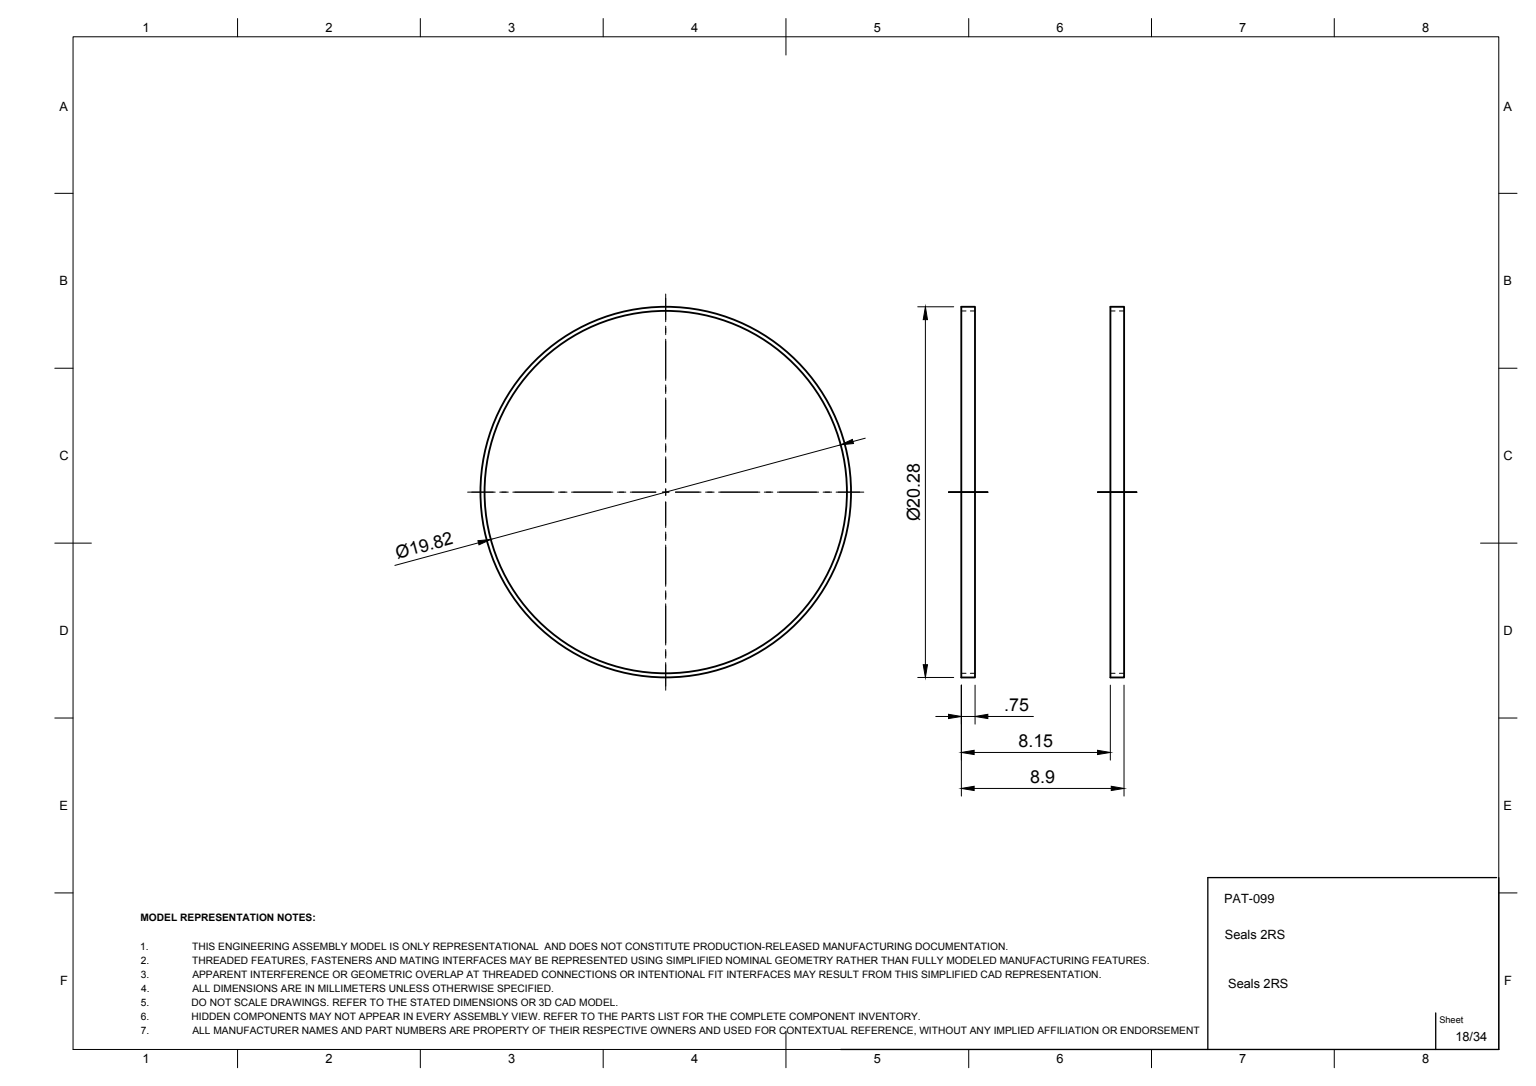
ISO-10303-21;
HEADER;
/* Generated by software containing ST-Developer
 * from STEP Tools, Inc. (www.steptools.com) 
 */

FILE_DESCRIPTION(
/* description */ ('PAT-099'),
/* implementation_level */ '2;1');

FILE_NAME(
/* name */ 'Seals 2RS.step',
/* time_stamp */ '2026-10-29T17:25:42-07:00',
/* author */ (''),
/* organization */ (''),
/* preprocessor_version */ 'ST-DEVELOPER v20.2',
/* originating_system */ 'Autodesk Translation Framework v15.17.0.0',
/* authorisation */ '');

FILE_SCHEMA (('AUTOMOTIVE_DESIGN { 1 0 10303 214 3 1 1 }'));
ENDSEC;

DATA;
#10=MECHANICAL_DESIGN_GEOMETRIC_PRESENTATION_REPRESENTATION('',(#368,#369),#11035);
#311=SHAPE_REPRESENTATION_RELATIONSHIP('SRR','None',#11184,#336);
#336=ADVANCED_BREP_SHAPE_REPRESENTATION('',(#399,#400),#11034);
#368=STYLED_ITEM('',(#11386),#399);
#369=STYLED_ITEM('',(#11386),#400);
#399=MANIFOLD_SOLID_BREP('Body1',#4738);
#400=MANIFOLD_SOLID_BREP('Body2',#4739);
#519=FACE_BOUND('',#1332,.T.);
#520=FACE_BOUND('',#1335,.T.);
#521=FACE_BOUND('',#1338,.T.);
#522=FACE_BOUND('',#1341,.T.);
#655=PLANE('',#5615);
#656=PLANE('',#5620);
#657=PLANE('',#5623);
#658=PLANE('',#5628);
#932=FACE_OUTER_BOUND('',#1331,.T.);
#933=FACE_OUTER_BOUND('',#1333,.T.);
#934=FACE_OUTER_BOUND('',#1334,.T.);
#935=FACE_OUTER_BOUND('',#1336,.T.);
#936=FACE_OUTER_BOUND('',#1337,.T.);
#937=FACE_OUTER_BOUND('',#1339,.T.);
#938=FACE_OUTER_BOUND('',#1340,.T.);
#939=FACE_OUTER_BOUND('',#1342,.T.);
#1331=EDGE_LOOP('',(#4285));
#1332=EDGE_LOOP('',(#4286));
#1333=EDGE_LOOP('',(#4287,#4288,#4289,#4290));
#1334=EDGE_LOOP('',(#4291));
#1335=EDGE_LOOP('',(#4292));
#1336=EDGE_LOOP('',(#4293,#4294,#4295,#4296));
#1337=EDGE_LOOP('',(#4297));
#1338=EDGE_LOOP('',(#4298));
#1339=EDGE_LOOP('',(#4299,#4300,#4301,#4302));
#1340=EDGE_LOOP('',(#4303));
#1341=EDGE_LOOP('',(#4304));
#1342=EDGE_LOOP('',(#4305,#4306,#4307,#4308));
#1591=LINE('',#10913,#1843);
#1592=LINE('',#10918,#1844);
#1593=LINE('',#10927,#1845);
#1594=LINE('',#10932,#1846);
#1843=VECTOR('',#7124,1.013815);
#1844=VECTOR('',#7131,0.991185);
#1845=VECTOR('',#7142,1.013815);
#1846=VECTOR('',#7149,0.991185);
#2130=CIRCLE('',#5616,1.013815);
#2131=CIRCLE('',#5617,0.991185);
#2132=CIRCLE('',#5619,1.013815);
#2133=CIRCLE('',#5621,0.991185);
#2134=CIRCLE('',#5624,1.013815);
#2135=CIRCLE('',#5625,0.991185);
#2136=CIRCLE('',#5627,1.013815);
#2137=CIRCLE('',#5629,0.991185);
#2534=VERTEX_POINT('',#10906);
#2535=VERTEX_POINT('',#10908);
#2536=VERTEX_POINT('',#10911);
#2537=VERTEX_POINT('',#10915);
#2538=VERTEX_POINT('',#10920);
#2539=VERTEX_POINT('',#10922);
#2540=VERTEX_POINT('',#10925);
#2541=VERTEX_POINT('',#10929);
#3119=EDGE_CURVE('',#2534,#2534,#2130,.T.);
#3120=EDGE_CURVE('',#2535,#2535,#2131,.T.);
#3121=EDGE_CURVE('',#2536,#2536,#2132,.T.);
#3122=EDGE_CURVE('',#2536,#2534,#1591,.T.);
#3123=EDGE_CURVE('',#2537,#2537,#2133,.T.);
#3124=EDGE_CURVE('',#2537,#2535,#1592,.T.);
#3125=EDGE_CURVE('',#2538,#2538,#2134,.T.);
#3126=EDGE_CURVE('',#2539,#2539,#2135,.T.);
#3127=EDGE_CURVE('',#2540,#2540,#2136,.T.);
#3128=EDGE_CURVE('',#2540,#2538,#1593,.T.);
#3129=EDGE_CURVE('',#2541,#2541,#2137,.T.);
#3130=EDGE_CURVE('',#2541,#2539,#1594,.T.);
#4285=ORIENTED_EDGE('',*,*,#3119,.F.);
#4286=ORIENTED_EDGE('',*,*,#3120,.T.);
#4287=ORIENTED_EDGE('',*,*,#3121,.F.);
#4288=ORIENTED_EDGE('',*,*,#3122,.T.);
#4289=ORIENTED_EDGE('',*,*,#3119,.T.);
#4290=ORIENTED_EDGE('',*,*,#3122,.F.);
#4291=ORIENTED_EDGE('',*,*,#3121,.T.);
#4292=ORIENTED_EDGE('',*,*,#3123,.F.);
#4293=ORIENTED_EDGE('',*,*,#3123,.T.);
#4294=ORIENTED_EDGE('',*,*,#3124,.T.);
#4295=ORIENTED_EDGE('',*,*,#3120,.F.);
#4296=ORIENTED_EDGE('',*,*,#3124,.F.);
#4297=ORIENTED_EDGE('',*,*,#3125,.F.);
#4298=ORIENTED_EDGE('',*,*,#3126,.T.);
#4299=ORIENTED_EDGE('',*,*,#3127,.F.);
#4300=ORIENTED_EDGE('',*,*,#3128,.T.);
#4301=ORIENTED_EDGE('',*,*,#3125,.T.);
#4302=ORIENTED_EDGE('',*,*,#3128,.F.);
#4303=ORIENTED_EDGE('',*,*,#3127,.T.);
#4304=ORIENTED_EDGE('',*,*,#3129,.F.);
#4305=ORIENTED_EDGE('',*,*,#3129,.T.);
#4306=ORIENTED_EDGE('',*,*,#3130,.T.);
#4307=ORIENTED_EDGE('',*,*,#3126,.F.);
#4308=ORIENTED_EDGE('',*,*,#3130,.F.);
#4420=CYLINDRICAL_SURFACE('',#5618,1.013815);
#4421=CYLINDRICAL_SURFACE('',#5622,0.991185);
#4422=CYLINDRICAL_SURFACE('',#5626,1.013815);
#4423=CYLINDRICAL_SURFACE('',#5630,0.991185);
#4697=ADVANCED_FACE('',(#932,#519),#655,.T.);
#4698=ADVANCED_FACE('',(#933),#4420,.T.);
#4699=ADVANCED_FACE('',(#934,#520),#656,.T.);
#4700=ADVANCED_FACE('',(#935),#4421,.F.);
#4701=ADVANCED_FACE('',(#936,#521),#657,.T.);
#4702=ADVANCED_FACE('',(#937),#4422,.T.);
#4703=ADVANCED_FACE('',(#938,#522),#658,.T.);
#4704=ADVANCED_FACE('',(#939),#4423,.F.);
#4738=CLOSED_SHELL('',(#4697,#4698,#4699,#4700));
#4739=CLOSED_SHELL('',(#4701,#4702,#4703,#4704));
#5614=AXIS2_PLACEMENT_3D('',#10904,#7112,#7113);
#5615=AXIS2_PLACEMENT_3D('',#10905,#7114,#7115);
#5616=AXIS2_PLACEMENT_3D('',#10907,#7116,#7117);
#5617=AXIS2_PLACEMENT_3D('',#10909,#7118,#7119);
#5618=AXIS2_PLACEMENT_3D('',#10910,#7120,#7121);
#5619=AXIS2_PLACEMENT_3D('',#10912,#7122,#7123);
#5620=AXIS2_PLACEMENT_3D('',#10914,#7125,#7126);
#5621=AXIS2_PLACEMENT_3D('',#10916,#7127,#7128);
#5622=AXIS2_PLACEMENT_3D('',#10917,#7129,#7130);
#5623=AXIS2_PLACEMENT_3D('',#10919,#7132,#7133);
#5624=AXIS2_PLACEMENT_3D('',#10921,#7134,#7135);
#5625=AXIS2_PLACEMENT_3D('',#10923,#7136,#7137);
#5626=AXIS2_PLACEMENT_3D('',#10924,#7138,#7139);
#5627=AXIS2_PLACEMENT_3D('',#10926,#7140,#7141);
#5628=AXIS2_PLACEMENT_3D('',#10928,#7143,#7144);
#5629=AXIS2_PLACEMENT_3D('',#10930,#7145,#7146);
#5630=AXIS2_PLACEMENT_3D('',#10931,#7147,#7148);
#7112=DIRECTION('axis',(0.,0.,1.));
#7113=DIRECTION('refdir',(1.,0.,0.));
#7114=DIRECTION('center_axis',(0.,1.,0.));
#7115=DIRECTION('ref_axis',(0.,0.,1.));
#7116=DIRECTION('center_axis',(0.,-1.,0.));
#7117=DIRECTION('ref_axis',(1.,0.,0.));
#7118=DIRECTION('center_axis',(0.,-1.,0.));
#7119=DIRECTION('ref_axis',(1.,0.,0.));
#7120=DIRECTION('center_axis',(0.,-1.,0.));
#7121=DIRECTION('ref_axis',(1.,0.,0.));
#7122=DIRECTION('center_axis',(0.,-1.,0.));
#7123=DIRECTION('ref_axis',(1.,0.,0.));
#7124=DIRECTION('',(0.,1.,0.));
#7125=DIRECTION('center_axis',(0.,-1.,0.));
#7126=DIRECTION('ref_axis',(0.,0.,-1.));
#7127=DIRECTION('center_axis',(0.,-1.,0.));
#7128=DIRECTION('ref_axis',(1.,0.,0.));
#7129=DIRECTION('center_axis',(0.,-1.,0.));
#7130=DIRECTION('ref_axis',(1.,0.,0.));
#7131=DIRECTION('',(0.,1.,0.));
#7132=DIRECTION('center_axis',(0.,1.,0.));
#7133=DIRECTION('ref_axis',(0.,0.,1.));
#7134=DIRECTION('center_axis',(0.,-1.,0.));
#7135=DIRECTION('ref_axis',(1.,0.,0.));
#7136=DIRECTION('center_axis',(0.,-1.,0.));
#7137=DIRECTION('ref_axis',(1.,0.,0.));
#7138=DIRECTION('center_axis',(0.,-1.,0.));
#7139=DIRECTION('ref_axis',(1.,0.,0.));
#7140=DIRECTION('center_axis',(0.,-1.,0.));
#7141=DIRECTION('ref_axis',(1.,0.,0.));
#7142=DIRECTION('',(0.,1.,0.));
#7143=DIRECTION('center_axis',(0.,-1.,0.));
#7144=DIRECTION('ref_axis',(0.,0.,-1.));
#7145=DIRECTION('center_axis',(0.,-1.,0.));
#7146=DIRECTION('ref_axis',(1.,0.,0.));
#7147=DIRECTION('center_axis',(0.,-1.,0.));
#7148=DIRECTION('ref_axis',(1.,0.,0.));
#7149=DIRECTION('',(0.,1.,0.));
#10904=CARTESIAN_POINT('',(0.,0.,0.));
#10905=CARTESIAN_POINT('Origin',(1.013815,0.445,0.));
#10906=CARTESIAN_POINT('',(-1.013815,0.445,-1.24156529467757E-16));
#10907=CARTESIAN_POINT('Origin',(0.,0.445,0.));
#10908=CARTESIAN_POINT('',(-0.991185,0.445,-1.21385153761287E-16));
#10909=CARTESIAN_POINT('Origin',(0.,0.445,0.));
#10910=CARTESIAN_POINT('Origin',(0.,0.4075,0.));
#10911=CARTESIAN_POINT('',(-1.013815,0.37,-1.24156529467757E-16));
#10912=CARTESIAN_POINT('Origin',(0.,0.37,0.));
#10913=CARTESIAN_POINT('',(-1.013815,0.4075,-1.24156529467757E-16));
#10914=CARTESIAN_POINT('Origin',(0.991185,0.37,0.));
#10915=CARTESIAN_POINT('',(-0.991185,0.37,-1.21385153761287E-16));
#10916=CARTESIAN_POINT('Origin',(0.,0.37,0.));
#10917=CARTESIAN_POINT('Origin',(0.,0.4075,0.));
#10918=CARTESIAN_POINT('',(-0.991185,0.4075,-1.21385153761287E-16));
#10919=CARTESIAN_POINT('Origin',(1.013815,-0.37,0.));
#10920=CARTESIAN_POINT('',(-1.013815,-0.37,-1.24156529467757E-16));
#10921=CARTESIAN_POINT('Origin',(0.,-0.37,0.));
#10922=CARTESIAN_POINT('',(-0.991185,-0.37,-1.21385153761287E-16));
#10923=CARTESIAN_POINT('Origin',(0.,-0.37,0.));
#10924=CARTESIAN_POINT('Origin',(0.,-0.4075,0.));
#10925=CARTESIAN_POINT('',(-1.013815,-0.445,-1.24156529467757E-16));
#10926=CARTESIAN_POINT('Origin',(0.,-0.445,0.));
#10927=CARTESIAN_POINT('',(-1.013815,-0.4075,-1.24156529467757E-16));
#10928=CARTESIAN_POINT('Origin',(0.991185,-0.445,0.));
#10929=CARTESIAN_POINT('',(-0.991185,-0.445,-1.21385153761287E-16));
#10930=CARTESIAN_POINT('Origin',(0.,-0.445,0.));
#10931=CARTESIAN_POINT('Origin',(0.,-0.4075,0.));
#10932=CARTESIAN_POINT('',(-0.991185,-0.4075,-1.21385153761287E-16));
#11001=UNCERTAINTY_MEASURE_WITH_UNIT(LENGTH_MEASURE(0.001),#11036,
'DISTANCE_ACCURACY_VALUE',
'Maximum model space distance between geometric entities at asserted c
onnectivities');
#11002=UNCERTAINTY_MEASURE_WITH_UNIT(LENGTH_MEASURE(0.001),#11036,
'DISTANCE_ACCURACY_VALUE',
'Maximum model space distance between geometric entities at asserted c
onnectivities');
#11034=(
GEOMETRIC_REPRESENTATION_CONTEXT(3)
GLOBAL_UNCERTAINTY_ASSIGNED_CONTEXT((#11001))
GLOBAL_UNIT_ASSIGNED_CONTEXT((#11036,#11038,#11039))
REPRESENTATION_CONTEXT('','3D')
);
#11035=(
GEOMETRIC_REPRESENTATION_CONTEXT(3)
GLOBAL_UNCERTAINTY_ASSIGNED_CONTEXT((#11002))
GLOBAL_UNIT_ASSIGNED_CONTEXT((#11036,#11038,#11039))
REPRESENTATION_CONTEXT('','3D')
);
#11036=(
LENGTH_UNIT()
NAMED_UNIT(*)
SI_UNIT(.CENTI.,.METRE.)
);
#11038=(
NAMED_UNIT(*)
PLANE_ANGLE_UNIT()
SI_UNIT($,.RADIAN.)
);
#11039=(
NAMED_UNIT(*)
SI_UNIT($,.STERADIAN.)
SOLID_ANGLE_UNIT()
);
#11071=SHAPE_DEFINITION_REPRESENTATION(#11115,#11184);
#11115=PRODUCT_DEFINITION_SHAPE('',$,#11217);
#11184=SHAPE_REPRESENTATION('',(#5614),#11034);
#11185=PRODUCT_DEFINITION_CONTEXT('part definition',#11283,'design');
#11217=PRODUCT_DEFINITION('Seals 2RS','Seals 2RS',#11249,#11185);
#11249=PRODUCT_DEFINITION_FORMATION('',$,#11316);
#11283=APPLICATION_CONTEXT(
'Core Data for Automotive Mechanical Design Process');
#11284=PRODUCT_CONTEXT('part definition',#11283,'mechanical');
#11316=PRODUCT('Seals 2RS','Seals 2RS','Seals 2RS',(#11284));
#11380=COLOUR_RGB('Grey',0.48,0.52,0.57);
#11381=FILL_AREA_STYLE_COLOUR('',#11380);
#11382=FILL_AREA_STYLE('',(#11381));
#11383=SURFACE_STYLE_FILL_AREA(#11382);
#11384=SURFACE_SIDE_STYLE('',(#11383));
#11385=SURFACE_STYLE_USAGE(.BOTH.,#11384);
#11386=PRESENTATION_STYLE_ASSIGNMENT((#11385));
ENDSEC;
END-ISO-10303-21;
